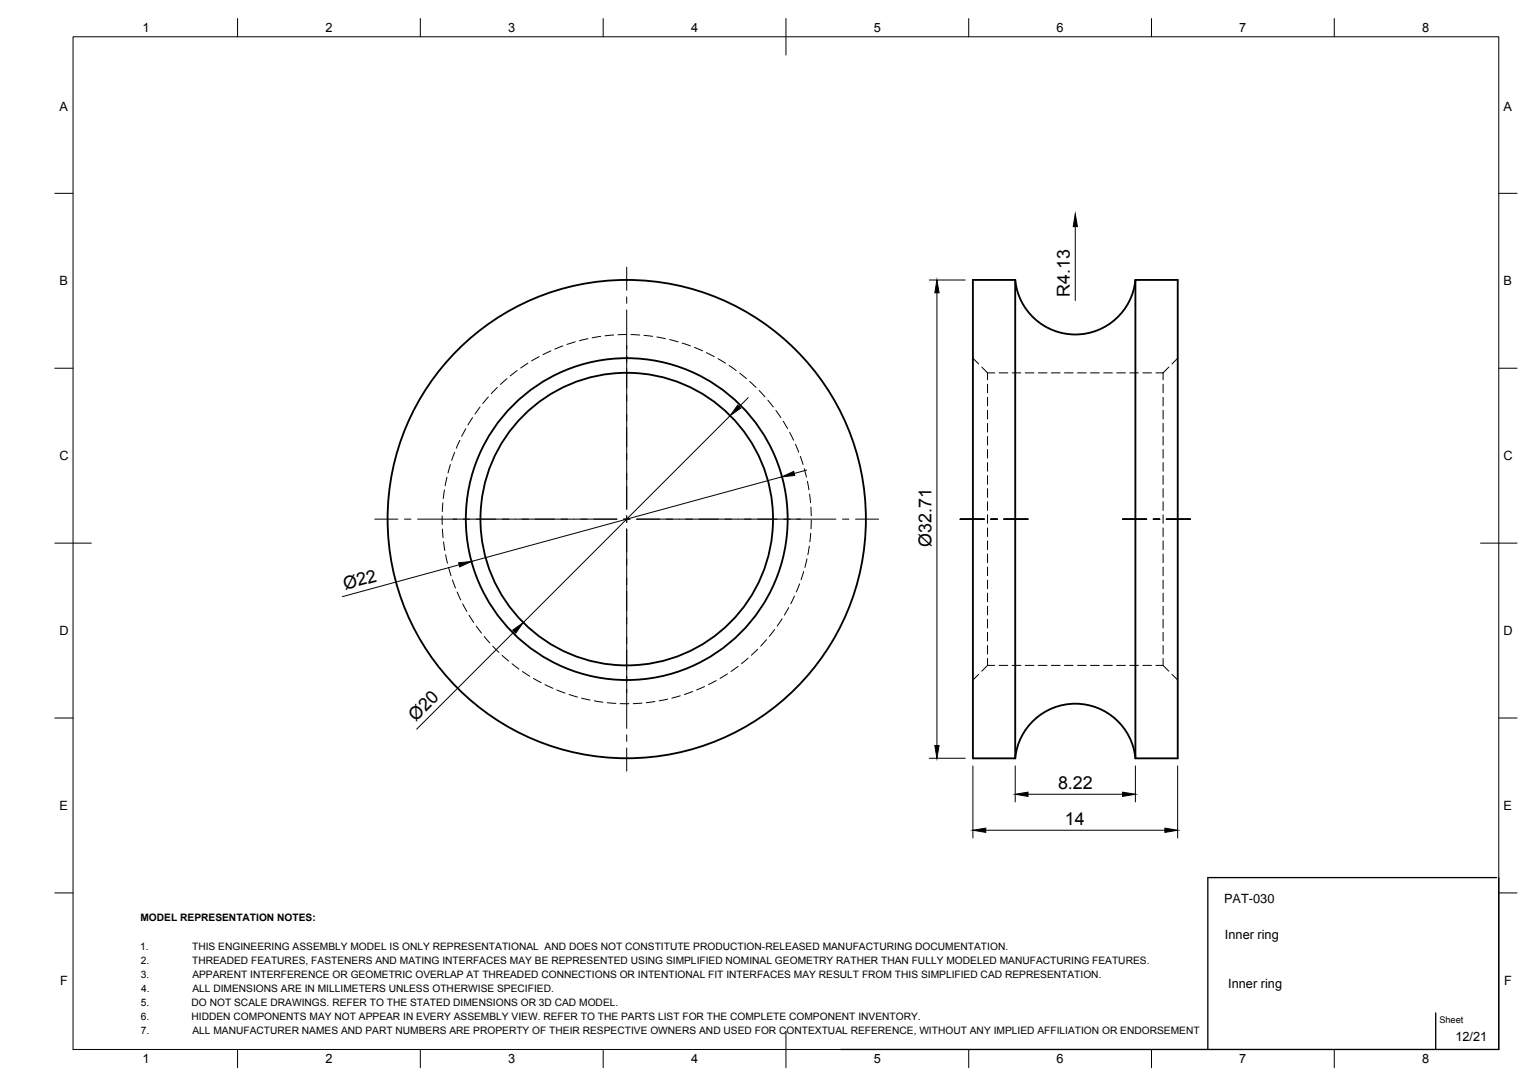
ISO-10303-21;
HEADER;
/* Generated by software containing ST-Developer
 * from STEP Tools, Inc. (www.steptools.com) 
 */

FILE_DESCRIPTION(
/* description */ ('Double-bearing flanged cartridge'),
/* implementation_level */ '2;1');

FILE_NAME(
/* name */ 'Inner ring.step',
/* time_stamp */ '2026-10-28T03:26:40-07:00',
/* author */ (''),
/* organization */ (''),
/* preprocessor_version */ 'ST-DEVELOPER v20.2',
/* originating_system */ 'Autodesk Translation Framework v15.17.0.0',
/* authorisation */ '');

FILE_SCHEMA (('AUTOMOTIVE_DESIGN { 1 0 10303 214 3 1 1 }'));
ENDSEC;

DATA;
#10=MECHANICAL_DESIGN_GEOMETRIC_PRESENTATION_REPRESENTATION('',(#191),#5535);
#152=CONICAL_SURFACE('',#2578,1.05,0.785398163397449);
#153=CONICAL_SURFACE('',#2585,1.05,0.785398163397449);
#160=TOROIDAL_SURFACE('',#2567,1.675,0.412776);
#163=SHAPE_REPRESENTATION_RELATIONSHIP('SRR','None',#5605,#177);
#177=ADVANCED_BREP_SHAPE_REPRESENTATION('',(#213),#5521);
#191=STYLED_ITEM('',(#5764),#213);
#213=MANIFOLD_SOLID_BREP('Body1',#2325);
#253=FACE_BOUND('',#563,.T.);
#254=FACE_BOUND('',#566,.T.);
#312=PLANE('',#2580);
#313=PLANE('',#2583);
#389=FACE_OUTER_BOUND('',#558,.T.);
#390=FACE_OUTER_BOUND('',#559,.T.);
#391=FACE_OUTER_BOUND('',#560,.T.);
#392=FACE_OUTER_BOUND('',#561,.T.);
#393=FACE_OUTER_BOUND('',#562,.T.);
#394=FACE_OUTER_BOUND('',#564,.T.);
#395=FACE_OUTER_BOUND('',#565,.T.);
#396=FACE_OUTER_BOUND('',#567,.T.);
#558=EDGE_LOOP('',(#1646,#1647,#1648,#1649,#1650,#1651));
#559=EDGE_LOOP('',(#1652,#1653,#1654,#1655,#1656));
#560=EDGE_LOOP('',(#1657,#1658,#1659,#1660));
#561=EDGE_LOOP('',(#1661,#1662,#1663,#1664));
#562=EDGE_LOOP('',(#1665));
#563=EDGE_LOOP('',(#1666));
#564=EDGE_LOOP('',(#1667,#1668,#1669,#1670,#1671));
#565=EDGE_LOOP('',(#1672));
#566=EDGE_LOOP('',(#1673));
#567=EDGE_LOOP('',(#1674,#1675,#1676,#1677));
#742=LINE('',#3808,#828);
#743=LINE('',#3814,#829);
#744=LINE('',#3818,#830);
#745=LINE('',#3824,#831);
#746=LINE('',#3829,#832);
#828=VECTOR('',#3027,1.63531);
#829=VECTOR('',#3034,1.);
#830=VECTOR('',#3039,1.05);
#831=VECTOR('',#3048,1.63531);
#832=VECTOR('',#3055,1.05);
#930=CIRCLE('',#2568,1.63531);
#931=CIRCLE('',#2569,1.63531);
#932=CIRCLE('',#2570,0.412776);
#933=CIRCLE('',#2571,1.63531);
#934=CIRCLE('',#2572,1.63531);
#935=CIRCLE('',#2574,1.63531);
#936=CIRCLE('',#2576,1.);
#937=CIRCLE('',#2577,1.);
#938=CIRCLE('',#2579,1.1);
#939=CIRCLE('',#2582,1.63531);
#940=CIRCLE('',#2584,1.1);
#1104=VERTEX_POINT('',#3797);
#1105=VERTEX_POINT('',#3798);
#1106=VERTEX_POINT('',#3801);
#1107=VERTEX_POINT('',#3803);
#1108=VERTEX_POINT('',#3807);
#1109=VERTEX_POINT('',#3811);
#1110=VERTEX_POINT('',#3813);
#1111=VERTEX_POINT('',#3817);
#1112=VERTEX_POINT('',#3822);
#1113=VERTEX_POINT('',#3826);
#1316=EDGE_CURVE('',#1104,#1105,#930,.T.);
#1317=EDGE_CURVE('',#1105,#1104,#931,.T.);
#1318=EDGE_CURVE('',#1105,#1106,#932,.T.);
#1319=EDGE_CURVE('',#1107,#1106,#933,.T.);
#1320=EDGE_CURVE('',#1106,#1107,#934,.T.);
#1321=EDGE_CURVE('',#1107,#1108,#742,.T.);
#1322=EDGE_CURVE('',#1108,#1108,#935,.T.);
#1323=EDGE_CURVE('',#1109,#1109,#936,.T.);
#1324=EDGE_CURVE('',#1109,#1110,#743,.T.);
#1325=EDGE_CURVE('',#1110,#1110,#937,.T.);
#1326=EDGE_CURVE('',#1110,#1111,#744,.T.);
#1327=EDGE_CURVE('',#1111,#1111,#938,.T.);
#1328=EDGE_CURVE('',#1112,#1112,#939,.T.);
#1329=EDGE_CURVE('',#1112,#1104,#745,.T.);
#1330=EDGE_CURVE('',#1113,#1113,#940,.T.);
#1331=EDGE_CURVE('',#1113,#1109,#746,.T.);
#1646=ORIENTED_EDGE('',*,*,#1316,.F.);
#1647=ORIENTED_EDGE('',*,*,#1317,.F.);
#1648=ORIENTED_EDGE('',*,*,#1318,.T.);
#1649=ORIENTED_EDGE('',*,*,#1319,.F.);
#1650=ORIENTED_EDGE('',*,*,#1320,.F.);
#1651=ORIENTED_EDGE('',*,*,#1318,.F.);
#1652=ORIENTED_EDGE('',*,*,#1319,.T.);
#1653=ORIENTED_EDGE('',*,*,#1320,.T.);
#1654=ORIENTED_EDGE('',*,*,#1321,.T.);
#1655=ORIENTED_EDGE('',*,*,#1322,.T.);
#1656=ORIENTED_EDGE('',*,*,#1321,.F.);
#1657=ORIENTED_EDGE('',*,*,#1323,.T.);
#1658=ORIENTED_EDGE('',*,*,#1324,.T.);
#1659=ORIENTED_EDGE('',*,*,#1325,.F.);
#1660=ORIENTED_EDGE('',*,*,#1324,.F.);
#1661=ORIENTED_EDGE('',*,*,#1325,.T.);
#1662=ORIENTED_EDGE('',*,*,#1326,.T.);
#1663=ORIENTED_EDGE('',*,*,#1327,.F.);
#1664=ORIENTED_EDGE('',*,*,#1326,.F.);
#1665=ORIENTED_EDGE('',*,*,#1322,.F.);
#1666=ORIENTED_EDGE('',*,*,#1327,.T.);
#1667=ORIENTED_EDGE('',*,*,#1328,.F.);
#1668=ORIENTED_EDGE('',*,*,#1329,.T.);
#1669=ORIENTED_EDGE('',*,*,#1316,.T.);
#1670=ORIENTED_EDGE('',*,*,#1317,.T.);
#1671=ORIENTED_EDGE('',*,*,#1329,.F.);
#1672=ORIENTED_EDGE('',*,*,#1328,.T.);
#1673=ORIENTED_EDGE('',*,*,#1330,.F.);
#1674=ORIENTED_EDGE('',*,*,#1330,.T.);
#1675=ORIENTED_EDGE('',*,*,#1331,.T.);
#1676=ORIENTED_EDGE('',*,*,#1323,.F.);
#1677=ORIENTED_EDGE('',*,*,#1331,.F.);
#2130=CYLINDRICAL_SURFACE('',#2573,1.63531);
#2131=CYLINDRICAL_SURFACE('',#2575,1.);
#2132=CYLINDRICAL_SURFACE('',#2581,1.63531);
#2203=ADVANCED_FACE('',(#389),#160,.F.);
#2204=ADVANCED_FACE('',(#390),#2130,.T.);
#2205=ADVANCED_FACE('',(#391),#2131,.F.);
#2206=ADVANCED_FACE('',(#392),#152,.F.);
#2207=ADVANCED_FACE('',(#393,#253),#312,.T.);
#2208=ADVANCED_FACE('',(#394),#2132,.T.);
#2209=ADVANCED_FACE('',(#395,#254),#313,.T.);
#2210=ADVANCED_FACE('',(#396),#153,.F.);
#2325=CLOSED_SHELL('',(#2203,#2204,#2205,#2206,#2207,#2208,#2209,#2210));
#2566=AXIS2_PLACEMENT_3D('',#3795,#3011,#3012);
#2567=AXIS2_PLACEMENT_3D('',#3796,#3013,#3014);
#2568=AXIS2_PLACEMENT_3D('',#3799,#3015,#3016);
#2569=AXIS2_PLACEMENT_3D('',#3800,#3017,#3018);
#2570=AXIS2_PLACEMENT_3D('',#3802,#3019,#3020);
#2571=AXIS2_PLACEMENT_3D('',#3804,#3021,#3022);
#2572=AXIS2_PLACEMENT_3D('',#3805,#3023,#3024);
#2573=AXIS2_PLACEMENT_3D('',#3806,#3025,#3026);
#2574=AXIS2_PLACEMENT_3D('',#3809,#3028,#3029);
#2575=AXIS2_PLACEMENT_3D('',#3810,#3030,#3031);
#2576=AXIS2_PLACEMENT_3D('',#3812,#3032,#3033);
#2577=AXIS2_PLACEMENT_3D('',#3815,#3035,#3036);
#2578=AXIS2_PLACEMENT_3D('',#3816,#3037,#3038);
#2579=AXIS2_PLACEMENT_3D('',#3819,#3040,#3041);
#2580=AXIS2_PLACEMENT_3D('',#3820,#3042,#3043);
#2581=AXIS2_PLACEMENT_3D('',#3821,#3044,#3045);
#2582=AXIS2_PLACEMENT_3D('',#3823,#3046,#3047);
#2583=AXIS2_PLACEMENT_3D('',#3825,#3049,#3050);
#2584=AXIS2_PLACEMENT_3D('',#3827,#3051,#3052);
#2585=AXIS2_PLACEMENT_3D('',#3828,#3053,#3054);
#3011=DIRECTION('axis',(0.,0.,1.));
#3012=DIRECTION('refdir',(1.,0.,0.));
#3013=DIRECTION('center_axis',(0.,-1.,0.));
#3014=DIRECTION('ref_axis',(0.,0.,-1.));
#3015=DIRECTION('center_axis',(0.,-1.,0.));
#3016=DIRECTION('ref_axis',(1.,0.,0.));
#3017=DIRECTION('center_axis',(0.,-1.,0.));
#3018=DIRECTION('ref_axis',(1.,0.,0.));
#3019=DIRECTION('center_axis',(1.,0.,1.22464679914735E-16));
#3020=DIRECTION('ref_axis',(-1.22464679914735E-16,0.,1.));
#3021=DIRECTION('center_axis',(0.,1.,0.));
#3022=DIRECTION('ref_axis',(1.,0.,0.));
#3023=DIRECTION('center_axis',(0.,1.,0.));
#3024=DIRECTION('ref_axis',(1.,0.,0.));
#3025=DIRECTION('center_axis',(0.,-1.,0.));
#3026=DIRECTION('ref_axis',(1.,0.,0.));
#3027=DIRECTION('',(0.,1.,0.));
#3028=DIRECTION('center_axis',(0.,-1.,0.));
#3029=DIRECTION('ref_axis',(1.,0.,0.));
#3030=DIRECTION('center_axis',(0.,-1.,0.));
#3031=DIRECTION('ref_axis',(1.,0.,0.));
#3032=DIRECTION('center_axis',(0.,-1.,0.));
#3033=DIRECTION('ref_axis',(1.,0.,0.));
#3034=DIRECTION('',(0.,1.,0.));
#3035=DIRECTION('center_axis',(0.,-1.,0.));
#3036=DIRECTION('ref_axis',(1.,0.,0.));
#3037=DIRECTION('center_axis',(0.,1.,0.));
#3038=DIRECTION('ref_axis',(1.,0.,0.));
#3039=DIRECTION('',(-0.707106781186548,0.707106781186547,-8.65956056235494E-17));
#3040=DIRECTION('center_axis',(0.,-1.,0.));
#3041=DIRECTION('ref_axis',(1.,0.,0.));
#3042=DIRECTION('center_axis',(0.,1.,0.));
#3043=DIRECTION('ref_axis',(0.,0.,1.));
#3044=DIRECTION('center_axis',(0.,-1.,0.));
#3045=DIRECTION('ref_axis',(1.,0.,0.));
#3046=DIRECTION('center_axis',(0.,-1.,0.));
#3047=DIRECTION('ref_axis',(1.,0.,0.));
#3048=DIRECTION('',(0.,1.,0.));
#3049=DIRECTION('center_axis',(0.,-1.,0.));
#3050=DIRECTION('ref_axis',(0.,0.,-1.));
#3051=DIRECTION('center_axis',(0.,-1.,0.));
#3052=DIRECTION('ref_axis',(1.,0.,0.));
#3053=DIRECTION('center_axis',(0.,-1.,0.));
#3054=DIRECTION('ref_axis',(1.,0.,0.));
#3055=DIRECTION('',(0.707106781186548,0.707106781186547,8.65956056235494E-17));
#3795=CARTESIAN_POINT('',(0.,0.,0.));
#3796=CARTESIAN_POINT('Origin',(0.,0.,0.));
#3797=CARTESIAN_POINT('',(-1.63531,-0.410863395882378,-2.00267715711366E-16));
#3798=CARTESIAN_POINT('',(-2.00267715711366E-16,-0.410863395882378,1.63531));
#3799=CARTESIAN_POINT('Origin',(0.,-0.410863395882378,0.));
#3800=CARTESIAN_POINT('Origin',(0.,-0.410863395882378,0.));
#3801=CARTESIAN_POINT('',(-2.00267715711366E-16,0.410863395882378,1.63531));
#3802=CARTESIAN_POINT('Origin',(-2.05128338857182E-16,0.,1.675));
#3803=CARTESIAN_POINT('',(-1.63531,0.410863395882378,2.00267715711366E-16));
#3804=CARTESIAN_POINT('Origin',(0.,0.410863395882378,0.));
#3805=CARTESIAN_POINT('Origin',(0.,0.410863395882378,0.));
#3806=CARTESIAN_POINT('Origin',(0.,0.,0.));
#3807=CARTESIAN_POINT('',(-1.63531,0.7,-2.00267715711366E-16));
#3808=CARTESIAN_POINT('',(-1.63531,0.,-2.00267715711366E-16));
#3809=CARTESIAN_POINT('Origin',(0.,0.7,0.));
#3810=CARTESIAN_POINT('Origin',(0.,0.,0.));
#3811=CARTESIAN_POINT('',(-1.,-0.6,-1.22464679914735E-16));
#3812=CARTESIAN_POINT('Origin',(0.,-0.6,0.));
#3813=CARTESIAN_POINT('',(-1.,0.6,-1.22464679914735E-16));
#3814=CARTESIAN_POINT('',(-1.,0.,-1.22464679914735E-16));
#3815=CARTESIAN_POINT('Origin',(0.,0.6,0.));
#3816=CARTESIAN_POINT('Origin',(0.,0.65,0.));
#3817=CARTESIAN_POINT('',(-1.1,0.7,-1.34711147906209E-16));
#3818=CARTESIAN_POINT('',(-1.05,0.65,-1.28587913910472E-16));
#3819=CARTESIAN_POINT('Origin',(0.,0.7,0.));
#3820=CARTESIAN_POINT('Origin',(1.63531,0.7,0.));
#3821=CARTESIAN_POINT('Origin',(0.,0.,0.));
#3822=CARTESIAN_POINT('',(-1.63531,-0.7,-2.00267715711366E-16));
#3823=CARTESIAN_POINT('Origin',(0.,-0.7,0.));
#3824=CARTESIAN_POINT('',(-1.63531,0.,-2.00267715711366E-16));
#3825=CARTESIAN_POINT('Origin',(1.1,-0.7,0.));
#3826=CARTESIAN_POINT('',(-1.1,-0.7,-1.34711147906209E-16));
#3827=CARTESIAN_POINT('Origin',(0.,-0.7,0.));
#3828=CARTESIAN_POINT('Origin',(0.,-0.65,0.));
#3829=CARTESIAN_POINT('',(-1.05,-0.65,-1.28587913910472E-16));
#5502=UNCERTAINTY_MEASURE_WITH_UNIT(LENGTH_MEASURE(0.001),#5536,
'DISTANCE_ACCURACY_VALUE',
'Maximum model space distance between geometric entities at asserted c
onnectivities');
#5516=UNCERTAINTY_MEASURE_WITH_UNIT(LENGTH_MEASURE(0.001),#5536,
'DISTANCE_ACCURACY_VALUE',
'Maximum model space distance between geometric entities at asserted c
onnectivities');
#5521=(
GEOMETRIC_REPRESENTATION_CONTEXT(3)
GLOBAL_UNCERTAINTY_ASSIGNED_CONTEXT((#5502))
GLOBAL_UNIT_ASSIGNED_CONTEXT((#5536,#5538,#5539))
REPRESENTATION_CONTEXT('','3D')
);
#5535=(
GEOMETRIC_REPRESENTATION_CONTEXT(3)
GLOBAL_UNCERTAINTY_ASSIGNED_CONTEXT((#5516))
GLOBAL_UNIT_ASSIGNED_CONTEXT((#5536,#5538,#5539))
REPRESENTATION_CONTEXT('','3D')
);
#5536=(
LENGTH_UNIT()
NAMED_UNIT(*)
SI_UNIT(.CENTI.,.METRE.)
);
#5538=(
NAMED_UNIT(*)
PLANE_ANGLE_UNIT()
SI_UNIT($,.RADIAN.)
);
#5539=(
NAMED_UNIT(*)
SI_UNIT($,.STERADIAN.)
SOLID_ANGLE_UNIT()
);
#5544=SHAPE_DEFINITION_REPRESENTATION(#5562,#5605);
#5562=PRODUCT_DEFINITION_SHAPE('',$,#5624);
#5605=SHAPE_REPRESENTATION('',(#2566),#5521);
#5619=PRODUCT_DEFINITION_CONTEXT('part definition',#5675,'design');
#5624=PRODUCT_DEFINITION('Inner ring','Inner ring',#5642,#5619);
#5642=PRODUCT_DEFINITION_FORMATION('',$,#5681);
#5675=APPLICATION_CONTEXT(
'Core Data for Automotive Mechanical Design Process');
#5676=PRODUCT_CONTEXT('part definition',#5675,'mechanical');
#5681=PRODUCT('Inner ring','Inner ring','Inner ring',(#5676));
#5758=COLOUR_RGB('Grey',0.48,0.52,0.57);
#5759=FILL_AREA_STYLE_COLOUR('',#5758);
#5760=FILL_AREA_STYLE('',(#5759));
#5761=SURFACE_STYLE_FILL_AREA(#5760);
#5762=SURFACE_SIDE_STYLE('',(#5761));
#5763=SURFACE_STYLE_USAGE(.BOTH.,#5762);
#5764=PRESENTATION_STYLE_ASSIGNMENT((#5763));
ENDSEC;
END-ISO-10303-21;
